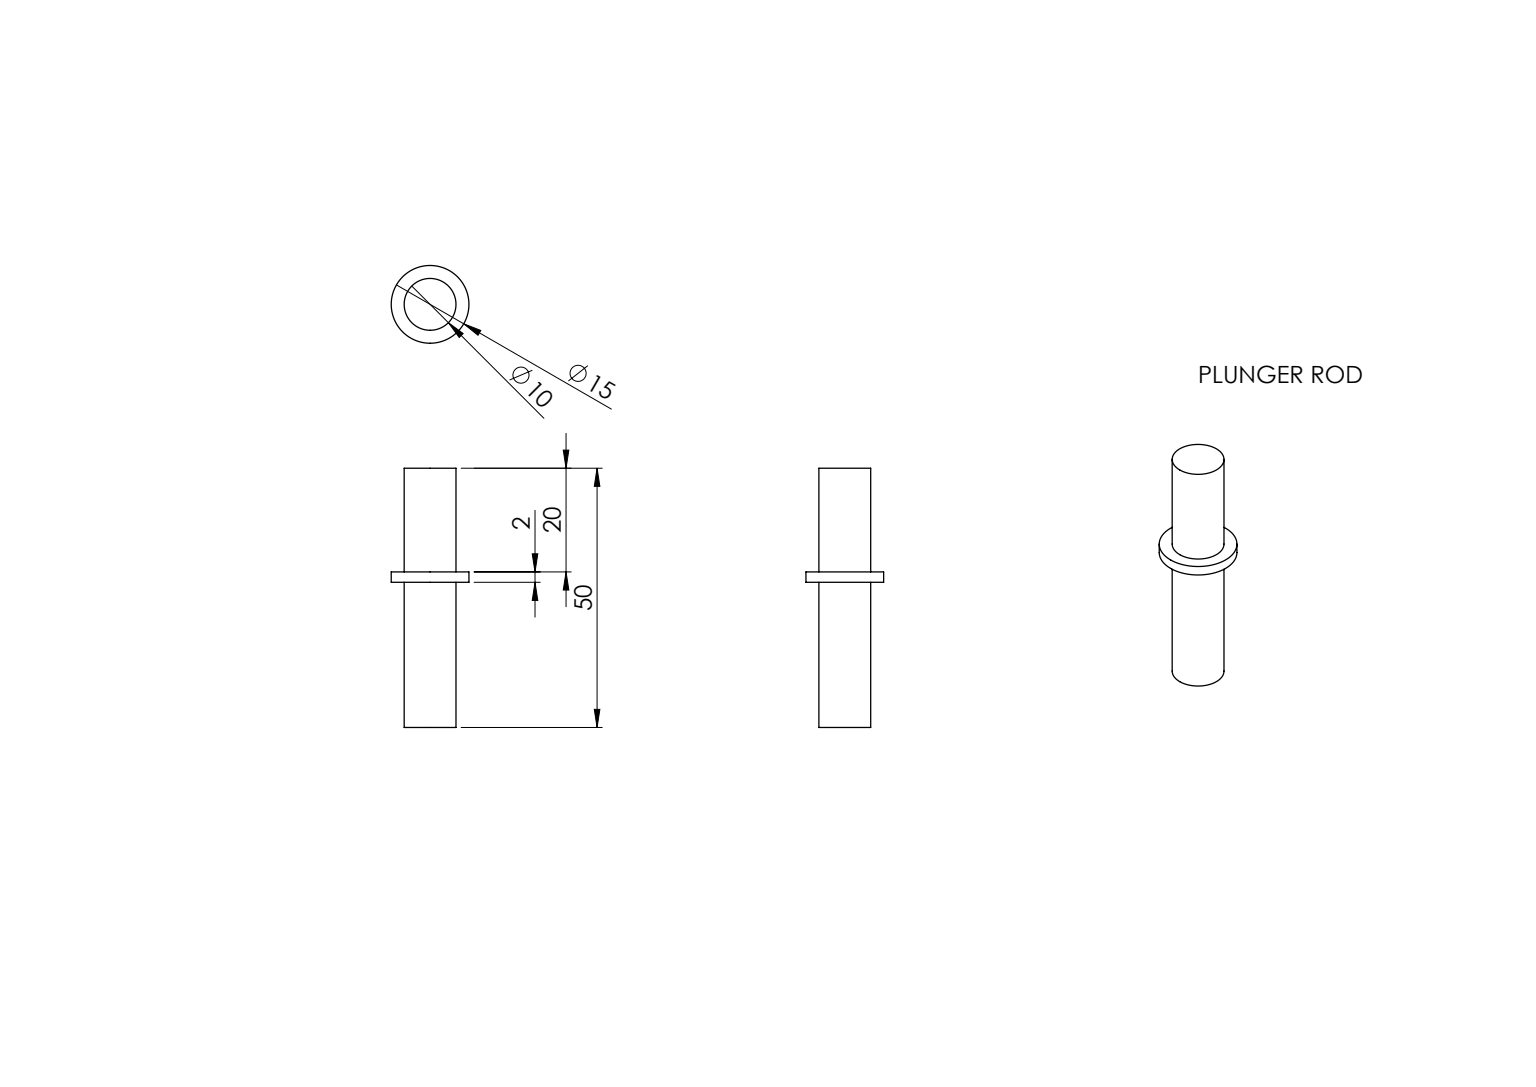
ISO-10303-21;
HEADER;
FILE_DESCRIPTION (('STEP AP214'),
    '1' );
FILE_NAME ('plunger rod.step',
    '2026-10-27T14:18:53',
    ( '' ),
    ( '' ),
    'SwSTEP 2.0',
    'SolidWorks 2026',
    '' );
FILE_SCHEMA (( 'AUTOMOTIVE_DESIGN' ));
ENDSEC;

DATA;
#51=VERTEX_POINT ( 'NONE', #4696 ) ;
#83=DIRECTION ( 'NONE',  ( 0.000000000000000000, 1.000000000000000000, 0.000000000000000000 ) ) ;
#108=AXIS2_PLACEMENT_3D ( 'NONE', #1468, #5154, #2894 ) ;
#114=FACE_OUTER_BOUND ( 'NONE', #3648, .T. ) ;
#118=VECTOR ( 'NONE', #5034, 1000.000000000000000 ) ;
#129=DIRECTION ( 'NONE',  ( -0.000000000000000000, -1.000000000000000000, -0.000000000000000000 ) ) ;
#152=DIRECTION ( 'NONE',  ( -0.000000000000000000, -1.000000000000000000, -0.000000000000000000 ) ) ;
#154=EDGE_LOOP ( 'NONE', ( #4564, #1318, #947, #4844 ) ) ;
#221=UNCERTAINTY_MEASURE_WITH_UNIT (LENGTH_MEASURE( 1.000000000000000082E-05 ), #1761, 'distance_accuracy_value', 'NONE');
#293=STYLED_ITEM('',(#6020),#2209);
#314=AXIS2_PLACEMENT_3D ( 'NONE', #3288, #1427, #2751 ) ;
#327=DIRECTION ( 'NONE',  ( 0.000000000000000000, 0.000000000000000000, 1.000000000000000000 ) ) ;
#373=FILL_AREA_STYLE ('',( #5951 ) ) ;
#407=CIRCLE ( 'NONE', #1166, 5.000000000000004441 ) ;
#408=FACE_BOUND ( 'NONE', #3152, .T. ) ;
#412=CIRCLE ( 'NONE', #978, 5.000000000000004441 ) ;
#419=DIRECTION ( 'NONE',  ( 0.000000000000000000, 1.000000000000000000, 0.000000000000000000 ) ) ;
#424=CARTESIAN_POINT ( 'NONE',  ( -45.00000000000001421, 50.00000000000000000, 50.00000000000000000 ) ) ;
#427=CYLINDRICAL_SURFACE ( 'NONE', #3498, 5.000000000000004441 ) ;
#470=ADVANCED_FACE ( 'NONE', ( #2397 ), #5641, .F. ) ;
#481=PRODUCT_DEFINITION_SHAPE ( 'NONE', 'NONE',  #3494 ) ;
#523=DIRECTION ( 'NONE',  ( 0.000000000000000000, -0.000000000000000000, 1.000000000000000000 ) ) ;
#532=DIRECTION ( 'NONE',  ( -0.000000000000000000, -1.000000000000000000, -0.000000000000000000 ) ) ;
#548=ORIENTED_EDGE ( 'NONE', *, *, #5422, .F. ) ;
#564=FACE_OUTER_BOUND ( 'NONE', #4940, .T. ) ;
#583=FACE_OUTER_BOUND ( 'NONE', #5588, .T. ) ;
#610=ORIENTED_EDGE ( 'NONE', *, *, #5795, .F. ) ;
#623=FACE_OUTER_BOUND ( 'NONE', #2477, .T. ) ;
#624=CARTESIAN_POINT ( 'NONE',  ( -45.00000000000001421, 50.00000000000000000, 50.00000000000000000 ) ) ;
#667=DIRECTION ( 'NONE',  ( 1.000000000000000000, 0.000000000000000000, 0.000000000000000000 ) ) ;
#673=EDGE_CURVE ( 'NONE', #771, #4908, #3765, .T. ) ;
#701=VECTOR ( 'NONE', #83, 1000.000000000000000 ) ;
#713=EDGE_LOOP ( 'NONE', ( #4575, #4451 ) ) ;
#714=DIRECTION ( 'NONE',  ( 0.000000000000000000, 1.000000000000000000, 0.000000000000000000 ) ) ;
#764=VERTEX_POINT ( 'NONE', #4131 ) ;
#769=CARTESIAN_POINT ( 'NONE',  ( -45.00000000000001421, 30.00000000000000355, 45.00000000000000000 ) ) ;
#771=VERTEX_POINT ( 'NONE', #881 ) ;
#832=DIRECTION ( 'NONE',  ( 0.000000000000000000, 1.000000000000000000, 0.000000000000000000 ) ) ;
#848=ORIENTED_EDGE ( 'NONE', *, *, #3434, .T. ) ;
#866=DIRECTION ( 'NONE',  ( 0.000000000000000000, 1.000000000000000000, 0.000000000000000000 ) ) ;
#877=ORIENTED_EDGE ( 'NONE', *, *, #1717, .F. ) ;
#878=CARTESIAN_POINT ( 'NONE',  ( -45.00000000000001421, 50.00000000000000000, 39.99999999999999289 ) ) ;
#881=CARTESIAN_POINT ( 'NONE',  ( -45.00000000000001421, 30.00000000000000355, 39.99999999999999289 ) ) ;
#884=CARTESIAN_POINT ( 'NONE',  ( -45.00000000000001421, 30.00000000000000355, 45.00000000000000000 ) ) ;
#886=ORIENTED_EDGE ( 'NONE', *, *, #4132, .T. ) ;
#892=AXIS2_PLACEMENT_3D ( 'NONE', #1880, #1055, #2826 ) ;
#906=EDGE_CURVE ( 'NONE', #51, #2642, #3817, .T. ) ;
#947=ORIENTED_EDGE ( 'NONE', *, *, #3173, .T. ) ;
#959=CIRCLE ( 'NONE', #1734, 5.000000000000004441 ) ;
#978=AXIS2_PLACEMENT_3D ( 'NONE', #3629, #419, #3737 ) ;
#987=LINE ( 'NONE', #4700, #1564 ) ;
#1055=DIRECTION ( 'NONE',  ( 0.000000000000000000, 1.000000000000000000, 0.000000000000000000 ) ) ;
#1078=DIRECTION ( 'NONE',  ( 0.000000000000000000, 1.000000000000000000, 0.000000000000000000 ) ) ;
#1094=DIRECTION ( 'NONE',  ( 0.000000000000000000, 1.000000000000000000, 0.000000000000000000 ) ) ;
#1145=CARTESIAN_POINT ( 'NONE',  ( -45.00000000000001421, 28.00000000000000355, 45.00000000000000000 ) ) ;
#1161=CIRCLE ( 'NONE', #108, 5.000000000000004441 ) ;
#1166=AXIS2_PLACEMENT_3D ( 'NONE', #769, #1684, #327 ) ;
#1214=CARTESIAN_POINT ( 'NONE',  ( -45.00000000000001421, 30.00000000000000355, 45.00000000000000000 ) ) ;
#1227=ORIENTED_EDGE ( 'NONE', *, *, #1696, .T. ) ;
#1228=SHAPE_DEFINITION_REPRESENTATION ( #481, #3184 ) ;
#1249=MECHANICAL_DESIGN_GEOMETRIC_PRESENTATION_REPRESENTATION('',(#293),#1840);
#1252=CARTESIAN_POINT ( 'NONE',  ( -45.00000000000001421, 28.00000000000000355, 45.00000000000000000 ) ) ;
#1271=AXIS2_PLACEMENT_3D ( 'NONE', #5723, #1078, #2449 ) ;
#1317=LINE ( 'NONE', #4517, #118 ) ;
#1318=ORIENTED_EDGE ( 'NONE', *, *, #3090, .T. ) ;
#1322=LINE ( 'NONE', #3635, #1361 ) ;
#1329=SURFACE_STYLE_USAGE ( .BOTH. , #4559 ) ;
#1361=VECTOR ( 'NONE', #5485, 1000.000000000000000 ) ;
#1381=ADVANCED_FACE ( 'NONE', ( #564 ), #3747, .T. ) ;
#1384=CYLINDRICAL_SURFACE ( 'NONE', #3216, 5.000000000000004441 ) ;
#1399=PRODUCT ( 'plunger rod', 'plunger rod', '', ( #3836 ) ) ;
#1424=CARTESIAN_POINT ( 'NONE',  ( -45.00000000000001421, 28.00000000000000355, 52.50000000000000000 ) ) ;
#1427=DIRECTION ( 'NONE',  ( 0.000000000000000000, 1.000000000000000000, 0.000000000000000000 ) ) ;
#1430=EDGE_LOOP ( 'NONE', ( #886, #1975, #2983, #4894 ) ) ;
#1436=VERTEX_POINT ( 'NONE', #3775 ) ;
#1468=CARTESIAN_POINT ( 'NONE',  ( -45.00000000000001421, 0.000000000000000000, 45.00000000000000000 ) ) ;
#1488=DIRECTION ( 'NONE',  ( 0.000000000000000000, 1.000000000000000000, 0.000000000000000000 ) ) ;
#1564=VECTOR ( 'NONE', #532, 1000.000000000000000 ) ;
#1580=COLOUR_RGB ( '',0.8941176470588234615, 0.8941176470588234615, 0.8941176470588234615 ) ;
#1585=VECTOR ( 'NONE', #129, 1000.000000000000000 ) ;
#1632=DIRECTION ( 'NONE',  ( 0.000000000000000000, 0.000000000000000000, -1.000000000000000000 ) ) ;
#1652=EDGE_LOOP ( 'NONE', ( #3751, #3779 ) ) ;
#1653=DIRECTION ( 'NONE',  ( 0.000000000000000000, -0.000000000000000000, 1.000000000000000000 ) ) ;
#1668=AXIS2_PLACEMENT_3D ( 'NONE', #2053, #152, #1632 ) ;
#1680=VERTEX_POINT ( 'NONE', #424 ) ;
#1684=DIRECTION ( 'NONE',  ( 0.000000000000000000, 1.000000000000000000, 0.000000000000000000 ) ) ;
#1696=EDGE_CURVE ( 'NONE', #1436, #764, #5512, .T. ) ;
#1717=EDGE_CURVE ( 'NONE', #2658, #5946, #2347, .T. ) ;
#1727=SURFACE_STYLE_FILL_AREA ( #373 ) ;
#1734=AXIS2_PLACEMENT_3D ( 'NONE', #1145, #1094, #2515 ) ;
#1760=AXIS2_PLACEMENT_3D ( 'NONE', #5478, #4690, #523 ) ;
#1761=( LENGTH_UNIT ( ) NAMED_UNIT ( * ) SI_UNIT ( .MILLI., .METRE. ) );
#1787=DIRECTION ( 'NONE',  ( 0.000000000000000000, 0.000000000000000000, 1.000000000000000000 ) ) ;
#1840=( GEOMETRIC_REPRESENTATION_CONTEXT ( 3 ) GLOBAL_UNCERTAINTY_ASSIGNED_CONTEXT ( ( #3846 ) ) GLOBAL_UNIT_ASSIGNED_CONTEXT ( ( #3319, #2371, #1883 ) ) REPRESENTATION_CONTEXT ( 'NONE', 'WORKASPACE' ) );
#1869=ORIENTED_EDGE ( 'NONE', *, *, #3434, .F. ) ;
#1880=CARTESIAN_POINT ( 'NONE',  ( -45.00000000000001421, 30.00000000000000355, 45.00000000000000000 ) ) ;
#1883=( NAMED_UNIT ( * ) SI_UNIT ( $, .STERADIAN. ) SOLID_ANGLE_UNIT ( ) );
#1906=ORIENTED_EDGE ( 'NONE', *, *, #4132, .F. ) ;
#1908=CARTESIAN_POINT ( 'NONE',  ( -45.00000000000001421, 0.000000000000000000, 45.00000000000000000 ) ) ;
#1945=CIRCLE ( 'NONE', #892, 7.500000000000000000 ) ;
#1975=ORIENTED_EDGE ( 'NONE', *, *, #5356, .T. ) ;
#2053=CARTESIAN_POINT ( 'NONE',  ( -45.00000000000001421, 50.00000000000000000, 45.00000000000000000 ) ) ;
#2075=FACE_BOUND ( 'NONE', #3051, .T. ) ;
#2076=DIRECTION ( 'NONE',  ( -0.000000000000000000, -1.000000000000000000, -0.000000000000000000 ) ) ;
#2108=AXIS2_PLACEMENT_3D ( 'NONE', #2629, #866, #5071 ) ;
#2125=CARTESIAN_POINT ( 'NONE',  ( -45.00000000000001421, 0.000000000000000000, 39.99999999999999289 ) ) ;
#2140=DIRECTION ( 'NONE',  ( 0.000000000000000000, 1.000000000000000000, 0.000000000000000000 ) ) ;
#2169=CARTESIAN_POINT ( 'NONE',  ( -45.00000000000001421, 28.00000000000000355, 50.00000000000000000 ) ) ;
#2209=MANIFOLD_SOLID_BREP ( 'Boss-Extrude2', #2762 ) ;
#2246=( NAMED_UNIT ( * ) SI_UNIT ( $, .STERADIAN. ) SOLID_ANGLE_UNIT ( ) );
#2250=FACE_OUTER_BOUND ( 'NONE', #3231, .T. ) ;
#2256=AXIS2_PLACEMENT_3D ( 'NONE', #4492, #2140, #5847 ) ;
#2347=CIRCLE ( 'NONE', #2256, 7.500000000000000000 ) ;
#2351=ADVANCED_FACE ( 'NONE', ( #583 ), #5770, .T. ) ;
#2371=( NAMED_UNIT ( * ) PLANE_ANGLE_UNIT ( ) SI_UNIT ( $, .RADIAN. ) );
#2385=AXIS2_PLACEMENT_3D ( 'NONE', #1908, #1488, #5258 ) ;
#2397=FACE_OUTER_BOUND ( 'NONE', #713, .T. ) ;
#2449=DIRECTION ( 'NONE',  ( 0.000000000000000000, 0.000000000000000000, 1.000000000000000000 ) ) ;
#2456=EDGE_CURVE ( 'NONE', #51, #4013, #959, .T. ) ;
#2477=EDGE_LOOP ( 'NONE', ( #1906, #877 ) ) ;
#2499=DIRECTION ( 'NONE',  ( 0.000000000000000000, -0.000000000000000000, 1.000000000000000000 ) ) ;
#2515=DIRECTION ( 'NONE',  ( 0.000000000000000000, 0.000000000000000000, 1.000000000000000000 ) ) ;
#2629=CARTESIAN_POINT ( 'NONE',  ( -45.00000000000001421, 30.00000000000000355, 45.00000000000000000 ) ) ;
#2642=VERTEX_POINT ( 'NONE', #2125 ) ;
#2658=VERTEX_POINT ( 'NONE', #3645 ) ;
#2720=AXIS2_PLACEMENT_3D ( 'NONE', #4391, #714, #1653 ) ;
#2751=DIRECTION ( 'NONE',  ( 0.000000000000000000, 0.000000000000000000, 1.000000000000000000 ) ) ;
#2759=CARTESIAN_POINT ( 'NONE',  ( -45.00000000000001421, 30.00000000000000355, 50.00000000000000000 ) ) ;
#2762=CLOSED_SHELL ( 'NONE', ( #4840, #3428, #5467, #3190, #470, #2351, #3280, #2792, #4172, #1381 ) ) ;
#2765=PRESENTATION_STYLE_ASSIGNMENT (( #1329 ) ) ;
#2792=ADVANCED_FACE ( 'NONE', ( #408, #2250 ), #5053, .T. ) ;
#2826=DIRECTION ( 'NONE',  ( 0.000000000000000000, 0.000000000000000000, 1.000000000000000000 ) ) ;
#2833=PLANE ( 'NONE',  #1760 ) ;
#2893=ORIENTED_EDGE ( 'NONE', *, *, #5879, .T. ) ;
#2894=DIRECTION ( 'NONE',  ( 0.000000000000000000, 0.000000000000000000, 1.000000000000000000 ) ) ;
#2901=DIRECTION ( 'NONE',  ( 0.000000000000000000, 0.000000000000000000, -1.000000000000000000 ) ) ;
#2962=APPLICATION_CONTEXT ( 'automotive_design' ) ;
#2972=ORIENTED_EDGE ( 'NONE', *, *, #1696, .F. ) ;
#2983=ORIENTED_EDGE ( 'NONE', *, *, #5879, .F. ) ;
#2988=DIRECTION ( 'NONE',  ( 0.000000000000000000, 0.000000000000000000, 1.000000000000000000 ) ) ;
#3000=ORIENTED_EDGE ( 'NONE', *, *, #5803, .T. ) ;
#3003=PRODUCT_DEFINITION_CONTEXT ( 'detailed design', #2962, 'design' ) ;
#3005=ORIENTED_EDGE ( 'NONE', *, *, #1717, .T. ) ;
#3016=AXIS2_PLACEMENT_3D ( 'NONE', #1252, #832, #3206 ) ;
#3020=VERTEX_POINT ( 'NONE', #4027 ) ;
#3048=EDGE_LOOP ( 'NONE', ( #5809, #4137, #848, #610 ) ) ;
#3051=EDGE_LOOP ( 'NONE', ( #4913, #5188 ) ) ;
#3070=DIRECTION ( 'NONE',  ( 0.000000000000000000, 0.000000000000000000, 1.000000000000000000 ) ) ;
#3090=EDGE_CURVE ( 'NONE', #4013, #3020, #1322, .T. ) ;
#3099=CARTESIAN_POINT ( 'NONE',  ( -45.00000000000001421, 0.000000000000000000, 45.00000000000000000 ) ) ;
#3152=EDGE_LOOP ( 'NONE', ( #4869, #1869 ) ) ;
#3173=EDGE_CURVE ( 'NONE', #3020, #2642, #1161, .T. ) ;
#3178=FACE_OUTER_BOUND ( 'NONE', #1430, .T. ) ;
#3184=SHAPE_REPRESENTATION ( 'plunger rod', ( #5080 ), #4591 ) ;
#3190=ADVANCED_FACE ( 'NONE', ( #114 ), #1384, .T. ) ;
#3206=DIRECTION ( 'NONE',  ( 0.000000000000000000, 0.000000000000000000, 1.000000000000000000 ) ) ;
#3216=AXIS2_PLACEMENT_3D ( 'NONE', #3804, #5655, #5122 ) ;
#3231=EDGE_LOOP ( 'NONE', ( #2893, #1227 ) ) ;
#3240=ORIENTED_EDGE ( 'NONE', *, *, #2456, .F. ) ;
#3280=ADVANCED_FACE ( 'NONE', ( #2075, #623 ), #3415, .F. ) ;
#3288=CARTESIAN_POINT ( 'NONE',  ( -45.00000000000001421, 28.00000000000000355, 45.00000000000000000 ) ) ;
#3306=AXIS2_PLACEMENT_3D ( 'NONE', #3380, #3446, #2988 ) ;
#3319=( LENGTH_UNIT ( ) NAMED_UNIT ( * ) SI_UNIT ( .MILLI., .METRE. ) );
#3341=ORIENTED_EDGE ( 'NONE', *, *, #5795, .T. ) ;
#3373=CARTESIAN_POINT ( 'NONE',  ( -45.00000000000001421, 28.00000000000000355, 45.00000000000000000 ) ) ;
#3380=CARTESIAN_POINT ( 'NONE',  ( -45.00000000000001421, 50.00000000000000000, 45.00000000000000000 ) ) ;
#3415=PLANE ( 'NONE',  #2720 ) ;
#3428=ADVANCED_FACE ( 'NONE', ( #3178 ), #5386, .T. ) ;
#3434=EDGE_CURVE ( 'NONE', #4908, #771, #407, .T. ) ;
#3446=DIRECTION ( 'NONE',  ( 0.000000000000000000, 1.000000000000000000, 0.000000000000000000 ) ) ;
#3484=AXIS2_PLACEMENT_3D ( 'NONE', #1214, #4010, #3070 ) ;
#3494=PRODUCT_DEFINITION ( 'UNKNOWN', '', #3526, #3003 ) ;
#3498=AXIS2_PLACEMENT_3D ( 'NONE', #4003, #4029, #3665 ) ;
#3517=( GEOMETRIC_REPRESENTATION_CONTEXT ( 3 ) GLOBAL_UNCERTAINTY_ASSIGNED_CONTEXT ( ( #3913 ) ) GLOBAL_UNIT_ASSIGNED_CONTEXT ( ( #4062, #5021, #4503 ) ) REPRESENTATION_CONTEXT ( 'NONE', 'WORKASPACE' ) );
#3526=PRODUCT_DEFINITION_FORMATION_WITH_SPECIFIED_SOURCE ( 'ANY', '', #1399, .NOT_KNOWN. ) ;
#3527=CARTESIAN_POINT ( 'NONE',  ( 0.000000000000000000, 0.000000000000000000, 0.000000000000000000 ) ) ;
#3548=FACE_OUTER_BOUND ( 'NONE', #3048, .T. ) ;
#3600=CIRCLE ( 'NONE', #314, 7.500000000000000000 ) ;
#3629=CARTESIAN_POINT ( 'NONE',  ( -45.00000000000001421, 28.00000000000000355, 45.00000000000000000 ) ) ;
#3635=CARTESIAN_POINT ( 'NONE',  ( -45.00000000000001421, 50.00000000000000000, 50.00000000000000000 ) ) ;
#3645=CARTESIAN_POINT ( 'NONE',  ( -45.00000000000001421, 28.00000000000000355, 37.50000000000000000 ) ) ;
#3648=EDGE_LOOP ( 'NONE', ( #3956, #3240, #4384, #4412 ) ) ;
#3665=DIRECTION ( 'NONE',  ( 0.000000000000000000, 0.000000000000000000, -1.000000000000000000 ) ) ;
#3668=ORIENTED_EDGE ( 'NONE', *, *, #5356, .F. ) ;
#3705=AXIS2_PLACEMENT_3D ( 'NONE', #3099, #4954, #1787 ) ;
#3737=DIRECTION ( 'NONE',  ( 0.000000000000000000, 0.000000000000000000, 1.000000000000000000 ) ) ;
#3747=CYLINDRICAL_SURFACE ( 'NONE', #4429, 5.000000000000004441 ) ;
#3751=ORIENTED_EDGE ( 'NONE', *, *, #5422, .T. ) ;
#3765=CIRCLE ( 'NONE', #3484, 5.000000000000004441 ) ;
#3769=LINE ( 'NONE', #4239, #701 ) ;
#3775=CARTESIAN_POINT ( 'NONE',  ( -45.00000000000001421, 30.00000000000000355, 37.50000000000000000 ) ) ;
#3779=ORIENTED_EDGE ( 'NONE', *, *, #3791, .T. ) ;
#3791=EDGE_CURVE ( 'NONE', #1680, #4352, #5915, .T. ) ;
#3804=CARTESIAN_POINT ( 'NONE',  ( -45.00000000000001421, 50.00000000000000000, 45.00000000000000000 ) ) ;
#3812=FACE_OUTER_BOUND ( 'NONE', #154, .T. ) ;
#3817=LINE ( 'NONE', #5250, #1585 ) ;
#3818=EDGE_CURVE ( 'NONE', #1680, #4908, #5229, .T. ) ;
#3836=PRODUCT_CONTEXT ( 'NONE', #5751, 'mechanical' ) ;
#3846=UNCERTAINTY_MEASURE_WITH_UNIT (LENGTH_MEASURE( 1.000000000000000082E-05 ), #3319, 'distance_accuracy_value', 'NONE');
#3872=CYLINDRICAL_SURFACE ( 'NONE', #1668, 5.000000000000004441 ) ;
#3885=CIRCLE ( 'NONE', #1271, 5.000000000000004441 ) ;
#3913=UNCERTAINTY_MEASURE_WITH_UNIT (LENGTH_MEASURE( 1.000000000000000082E-05 ), #4062, 'distance_accuracy_value', 'NONE');
#3956=ORIENTED_EDGE ( 'NONE', *, *, #3090, .F. ) ;
#4001=DIRECTION ( 'NONE',  ( 0.000000000000000000, 1.000000000000000000, 0.000000000000000000 ) ) ;
#4003=CARTESIAN_POINT ( 'NONE',  ( -45.00000000000001421, 50.00000000000000000, 45.00000000000000000 ) ) ;
#4010=DIRECTION ( 'NONE',  ( 0.000000000000000000, 1.000000000000000000, 0.000000000000000000 ) ) ;
#4013=VERTEX_POINT ( 'NONE', #2169 ) ;
#4027=CARTESIAN_POINT ( 'NONE',  ( -45.00000000000001421, 0.000000000000000000, 50.00000000000000000 ) ) ;
#4029=DIRECTION ( 'NONE',  ( -0.000000000000000000, -1.000000000000000000, -0.000000000000000000 ) ) ;
#4062=( LENGTH_UNIT ( ) NAMED_UNIT ( * ) SI_UNIT ( .MILLI., .METRE. ) );
#4081=VECTOR ( 'NONE', #2076, 1000.000000000000000 ) ;
#4131=CARTESIAN_POINT ( 'NONE',  ( -45.00000000000001421, 30.00000000000000355, 52.50000000000000000 ) ) ;
#4132=EDGE_CURVE ( 'NONE', #5946, #2658, #3600, .T. ) ;
#4133=EDGE_CURVE ( 'NONE', #4013, #51, #412, .T. ) ;
#4137=ORIENTED_EDGE ( 'NONE', *, *, #3818, .T. ) ;
#4157=( NAMED_UNIT ( * ) PLANE_ANGLE_UNIT ( ) SI_UNIT ( $, .RADIAN. ) );
#4172=ADVANCED_FACE ( 'NONE', ( #5586 ), #2833, .T. ) ;
#4189=DIRECTION ( 'NONE',  ( -0.000000000000000000, -1.000000000000000000, -0.000000000000000000 ) ) ;
#4196=MECHANICAL_DESIGN_GEOMETRIC_PRESENTATION_REPRESENTATION('',(#4682),#3517);
#4239=CARTESIAN_POINT ( 'NONE',  ( -45.00000000000001421, 28.00000000000000355, 52.50000000000000000 ) ) ;
#4289=CIRCLE ( 'NONE', #3705, 5.000000000000004441 ) ;
#4352=VERTEX_POINT ( 'NONE', #878 ) ;
#4353=EDGE_CURVE ( 'NONE', #2642, #3020, #4289, .T. ) ;
#4382=DIRECTION ( 'NONE',  ( 0.000000000000000000, 0.000000000000000000, 1.000000000000000000 ) ) ;
#4384=ORIENTED_EDGE ( 'NONE', *, *, #906, .T. ) ;
#4391=CARTESIAN_POINT ( 'NONE',  ( -45.00000000000001421, 28.00000000000000355, 45.00000000000000000 ) ) ;
#4412=ORIENTED_EDGE ( 'NONE', *, *, #4353, .T. ) ;
#4429=AXIS2_PLACEMENT_3D ( 'NONE', #5690, #4189, #2901 ) ;
#4451=ORIENTED_EDGE ( 'NONE', *, *, #3173, .F. ) ;
#4492=CARTESIAN_POINT ( 'NONE',  ( -45.00000000000001421, 28.00000000000000355, 45.00000000000000000 ) ) ;
#4503=( NAMED_UNIT ( * ) SI_UNIT ( $, .STERADIAN. ) SOLID_ANGLE_UNIT ( ) );
#4517=CARTESIAN_POINT ( 'NONE',  ( -45.00000000000001421, 28.00000000000000355, 37.50000000000000000 ) ) ;
#4559=SURFACE_SIDE_STYLE ('',( #1727 ) ) ;
#4564=ORIENTED_EDGE ( 'NONE', *, *, #4133, .F. ) ;
#4575=ORIENTED_EDGE ( 'NONE', *, *, #4353, .F. ) ;
#4591=( GEOMETRIC_REPRESENTATION_CONTEXT ( 3 ) GLOBAL_UNCERTAINTY_ASSIGNED_CONTEXT ( ( #221 ) ) GLOBAL_UNIT_ASSIGNED_CONTEXT ( ( #1761, #4157, #2246 ) ) REPRESENTATION_CONTEXT ( 'NONE', 'WORKASPACE' ) );
#4622=SHAPE_REPRESENTATION_RELATIONSHIP ( 'NONE' , 'NONE' ,  #3184, #4787 ) ;
#4682=STYLED_ITEM ( 'NONE', ( #2765 ), #4787 ) ;
#4690=DIRECTION ( 'NONE',  ( 0.000000000000000000, 1.000000000000000000, 0.000000000000000000 ) ) ;
#4696=CARTESIAN_POINT ( 'NONE',  ( -45.00000000000001421, 28.00000000000000355, 39.99999999999999289 ) ) ;
#4700=CARTESIAN_POINT ( 'NONE',  ( -45.00000000000001421, 50.00000000000000000, 39.99999999999999289 ) ) ;
#4787=ADVANCED_BREP_SHAPE_REPRESENTATION ( '', ( #2209, #5080 ), #4591 ) ;
#4831=DIRECTION ( 'NONE',  ( 0.000000000000000000, 0.000000000000000000, 1.000000000000000000 ) ) ;
#4840=ADVANCED_FACE ( 'NONE', ( #3548 ), #427, .T. ) ;
#4844=ORIENTED_EDGE ( 'NONE', *, *, #906, .F. ) ;
#4869=ORIENTED_EDGE ( 'NONE', *, *, #673, .F. ) ;
#4894=ORIENTED_EDGE ( 'NONE', *, *, #5803, .F. ) ;
#4908=VERTEX_POINT ( 'NONE', #2759 ) ;
#4913=ORIENTED_EDGE ( 'NONE', *, *, #2456, .T. ) ;
#4940=EDGE_LOOP ( 'NONE', ( #5763, #548, #3341, #5601 ) ) ;
#4954=DIRECTION ( 'NONE',  ( 0.000000000000000000, 1.000000000000000000, 0.000000000000000000 ) ) ;
#5021=( NAMED_UNIT ( * ) PLANE_ANGLE_UNIT ( ) SI_UNIT ( $, .RADIAN. ) );
#5034=DIRECTION ( 'NONE',  ( 0.000000000000000000, 1.000000000000000000, 0.000000000000000000 ) ) ;
#5053=PLANE ( 'NONE',  #5613 ) ;
#5071=DIRECTION ( 'NONE',  ( 0.000000000000000000, 0.000000000000000000, 1.000000000000000000 ) ) ;
#5080=AXIS2_PLACEMENT_3D ( 'NONE', #3527, #4831, #667 ) ;
#5122=DIRECTION ( 'NONE',  ( 0.000000000000000000, 0.000000000000000000, -1.000000000000000000 ) ) ;
#5154=DIRECTION ( 'NONE',  ( 0.000000000000000000, 1.000000000000000000, 0.000000000000000000 ) ) ;
#5188=ORIENTED_EDGE ( 'NONE', *, *, #4133, .T. ) ;
#5219=DIRECTION ( 'NONE',  ( 0.000000000000000000, 1.000000000000000000, 0.000000000000000000 ) ) ;
#5225=AXIS2_PLACEMENT_3D ( 'NONE', #3373, #5219, #4382 ) ;
#5229=LINE ( 'NONE', #624, #4081 ) ;
#5250=CARTESIAN_POINT ( 'NONE',  ( -45.00000000000001421, 50.00000000000000000, 39.99999999999999289 ) ) ;
#5258=DIRECTION ( 'NONE',  ( 0.000000000000000000, -0.000000000000000000, 1.000000000000000000 ) ) ;
#5356=EDGE_CURVE ( 'NONE', #2658, #1436, #1317, .T. ) ;
#5386=CYLINDRICAL_SURFACE ( 'NONE', #3016, 7.500000000000000000 ) ;
#5422=EDGE_CURVE ( 'NONE', #4352, #1680, #3885, .T. ) ;
#5467=ADVANCED_FACE ( 'NONE', ( #3812 ), #3872, .T. ) ;
#5478=CARTESIAN_POINT ( 'NONE',  ( -45.00000000000001421, 50.00000000000000000, 45.00000000000000000 ) ) ;
#5485=DIRECTION ( 'NONE',  ( -0.000000000000000000, -1.000000000000000000, -0.000000000000000000 ) ) ;
#5512=CIRCLE ( 'NONE', #2108, 7.500000000000000000 ) ;
#5586=FACE_OUTER_BOUND ( 'NONE', #1652, .T. ) ;
#5588=EDGE_LOOP ( 'NONE', ( #3668, #3005, #3000, #2972 ) ) ;
#5601=ORIENTED_EDGE ( 'NONE', *, *, #673, .T. ) ;
#5613=AXIS2_PLACEMENT_3D ( 'NONE', #884, #4001, #2499 ) ;
#5641=PLANE ( 'NONE',  #2385 ) ;
#5655=DIRECTION ( 'NONE',  ( -0.000000000000000000, -1.000000000000000000, -0.000000000000000000 ) ) ;
#5690=CARTESIAN_POINT ( 'NONE',  ( -45.00000000000001421, 50.00000000000000000, 45.00000000000000000 ) ) ;
#5723=CARTESIAN_POINT ( 'NONE',  ( -45.00000000000001421, 50.00000000000000000, 45.00000000000000000 ) ) ;
#5751=APPLICATION_CONTEXT ( 'automotive_design' ) ;
#5763=ORIENTED_EDGE ( 'NONE', *, *, #3818, .F. ) ;
#5770=CYLINDRICAL_SURFACE ( 'NONE', #5225, 7.500000000000000000 ) ;
#5795=EDGE_CURVE ( 'NONE', #4352, #771, #987, .T. ) ;
#5803=EDGE_CURVE ( 'NONE', #5946, #764, #3769, .T. ) ;
#5809=ORIENTED_EDGE ( 'NONE', *, *, #3791, .F. ) ;
#5847=DIRECTION ( 'NONE',  ( 0.000000000000000000, 0.000000000000000000, 1.000000000000000000 ) ) ;
#5879=EDGE_CURVE ( 'NONE', #764, #1436, #1945, .T. ) ;
#5915=CIRCLE ( 'NONE', #3306, 5.000000000000004441 ) ;
#5946=VERTEX_POINT ( 'NONE', #1424 ) ;
#5951=FILL_AREA_STYLE_COLOUR ( '', #1580 ) ;
#6014=COLOUR_RGB('Grey',0.48,0.52,0.57);
#6015=FILL_AREA_STYLE_COLOUR('',#6014);
#6016=FILL_AREA_STYLE('',(#6015));
#6017=SURFACE_STYLE_FILL_AREA(#6016);
#6018=SURFACE_SIDE_STYLE('',(#6017));
#6019=SURFACE_STYLE_USAGE(.BOTH.,#6018);
#6020=PRESENTATION_STYLE_ASSIGNMENT((#6019));
ENDSEC;
END-ISO-10303-21;
